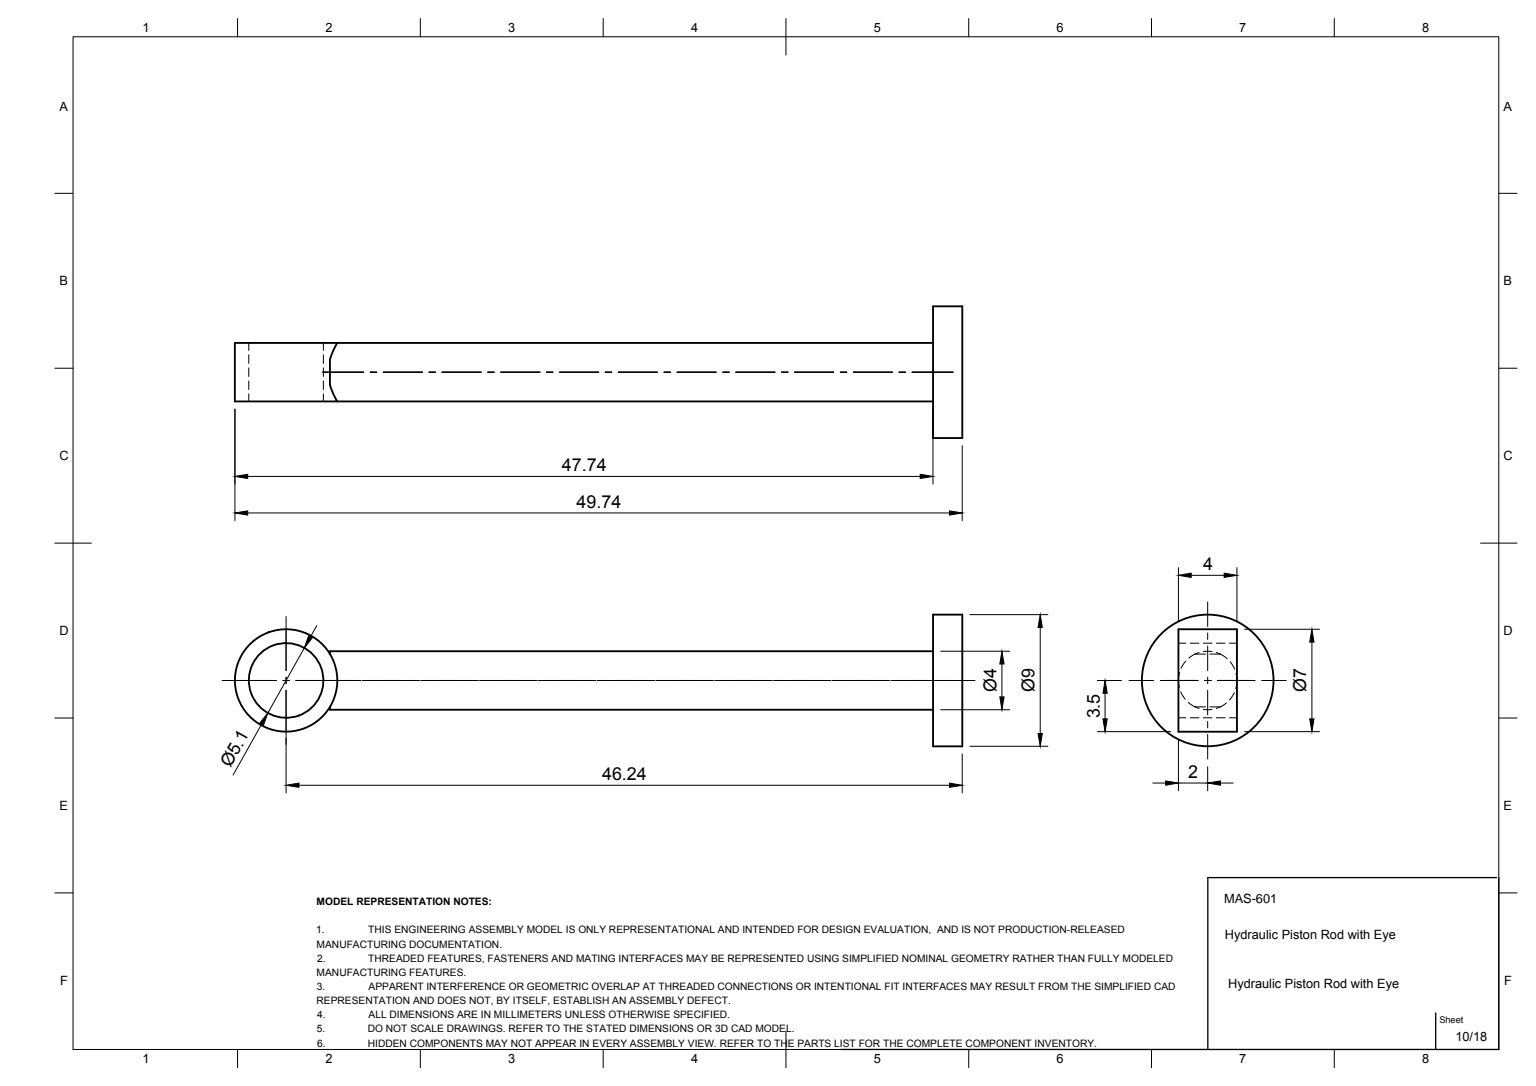
ISO-10303-21;
HEADER;
FILE_DESCRIPTION((''),'2;1');
FILE_NAME('Hydraulic Piston Rod with Eye.step','2026-10-06T07:37:42+05:00',(''),(''),'','','');
FILE_SCHEMA (('AUTOMOTIVE_DESIGN { 1 0 10303 214 3 1 1 }'));
ENDSEC;
DATA;
#10=MECHANICAL_DESIGN_GEOMETRIC_PRESENTATION_REPRESENTATION('',(#378),#18757);
#344=SHAPE_REPRESENTATION_RELATIONSHIP('SRR','None',#18862,#361) ;
#361=ADVANCED_BREP_SHAPE_REPRESENTATION('',(#395),#18745) ;
#378=STYLED_ITEM('',(#18956),#395) ;
#395=MANIFOLD_SOLID_BREP('Hydraulic Piston Rod with Eye',#9547) ;
#424=B_SPLINE_CURVE_WITH_KNOTS('',3,(#14684,#14685,#14686,#14687,#14688,
#14689,#14690,#14691),.UNSPECIFIED.,.F.,.F.,(4,2,2,4),(0.0875095450662273,
0.155297296869045,0.232550630259834,0.309803963650623),.UNSPECIFIED.) ;
#425=B_SPLINE_CURVE_WITH_KNOTS('',3,(#14695,#14696,#14697,#14698,#14699,
#14700,#14701,#14702),.UNSPECIFIED.,.F.,.F.,(4,2,2,4),(0.92941189095187,
1.00666522434266,1.08391855773345,1.15170630953627),.UNSPECIFIED.) ;
#426=B_SPLINE_CURVE_WITH_KNOTS('',3,(#14713,#14714,#14715,#14716,#14717,
#14718,#14719,#14720),.UNSPECIFIED.,.F.,.F.,(4,2,2,4),(0.707117472367471,
0.774905224170291,0.85215855756108,0.92941189095187),.UNSPECIFIED.) ;
#427=B_SPLINE_CURVE_WITH_KNOTS('',3,(#14723,#14724,#14725,#14726,#14727,
#14728,#14729,#14730),.UNSPECIFIED.,.F.,.F.,(4,2,2,4),(0.309803963650623,
0.387057297041413,0.464310630432203,0.532098382235022),.UNSPECIFIED.) ;
#569=CYLINDRICAL_SURFACE('',#10099,3.5) ;
#570=CYLINDRICAL_SURFACE('',#10102,2.55) ;
#571=CYLINDRICAL_SURFACE('',#10105,3.5) ;
#572=CYLINDRICAL_SURFACE('',#10115,2.) ;
#573=CYLINDRICAL_SURFACE('',#10119,4.50000000000001) ;
#717=FACE_BOUND('',#1868,.T.) ;
#718=FACE_BOUND('',#1870,.T.) ;
#719=FACE_BOUND('',#1875,.T.) ;
#862=PLANE('',#10108) ;
#863=PLANE('',#10109) ;
#864=PLANE('',#10110) ;
#865=PLANE('',#10113) ;
#866=PLANE('',#10117) ;
#867=PLANE('',#10121) ;
#1279=FACE_OUTER_BOUND('',#1864,.T.) ;
#1280=FACE_OUTER_BOUND('',#1865,.T.) ;
#1281=FACE_OUTER_BOUND('',#1866,.T.) ;
#1282=FACE_OUTER_BOUND('',#1867,.T.) ;
#1283=FACE_OUTER_BOUND('',#1869,.T.) ;
#1284=FACE_OUTER_BOUND('',#1871,.T.) ;
#1285=FACE_OUTER_BOUND('',#1872,.T.) ;
#1286=FACE_OUTER_BOUND('',#1873,.T.) ;
#1287=FACE_OUTER_BOUND('',#1874,.T.) ;
#1288=FACE_OUTER_BOUND('',#1876,.T.) ;
#1289=FACE_OUTER_BOUND('',#1877,.T.) ;
#1864=EDGE_LOOP('',(#7307,#7308,#7309,#7310,#7311,#7312)) ;
#1865=EDGE_LOOP('',(#7313,#7314,#7315,#7316)) ;
#1866=EDGE_LOOP('',(#7317,#7318,#7319,#7320,#7321,#7322)) ;
#1867=EDGE_LOOP('',(#7323,#7324)) ;
#1868=EDGE_LOOP('',(#7325)) ;
#1869=EDGE_LOOP('',(#7326,#7327)) ;
#1870=EDGE_LOOP('',(#7328)) ;
#1871=EDGE_LOOP('',(#7329,#7330,#7331)) ;
#1872=EDGE_LOOP('',(#7332,#7333)) ;
#1873=EDGE_LOOP('',(#7334,#7335,#7336,#7337,#7338,#7339,#7340,#7341,#7342,
#7343)) ;
#1874=EDGE_LOOP('',(#7344)) ;
#1875=EDGE_LOOP('',(#7345)) ;
#1876=EDGE_LOOP('',(#7346,#7347,#7348,#7349)) ;
#1877=EDGE_LOOP('',(#7350)) ;
#2545=LINE('',#14680,#3316) ;
#2546=LINE('',#14693,#3317) ;
#2547=LINE('',#14708,#3318) ;
#2548=LINE('',#14722,#3319) ;
#2549=LINE('',#14743,#3320) ;
#2550=LINE('',#14750,#3321) ;
#3316=VECTOR('',#11733,3.5) ;
#3317=VECTOR('',#11736,10.) ;
#3318=VECTOR('',#11743,2.55) ;
#3319=VECTOR('',#11750,10.) ;
#3320=VECTOR('',#11771,2.) ;
#3321=VECTOR('',#11780,4.50000000000001) ;
#3928=CIRCLE('',#10100,3.5) ;
#3929=CIRCLE('',#10101,3.5) ;
#3930=CIRCLE('',#10103,2.55) ;
#3931=CIRCLE('',#10104,2.55) ;
#3932=CIRCLE('',#10106,3.5) ;
#3933=CIRCLE('',#10107,3.5) ;
#3934=CIRCLE('',#10111,2.) ;
#3935=CIRCLE('',#10112,2.) ;
#3936=CIRCLE('',#10114,2.) ;
#3937=CIRCLE('',#10116,2.) ;
#3938=CIRCLE('',#10118,4.50000000000001) ;
#3939=CIRCLE('',#10120,4.50000000000001) ;
#4466=VERTEX_POINT('',#14678) ;
#4467=VERTEX_POINT('',#14679) ;
#4468=VERTEX_POINT('',#14681) ;
#4469=VERTEX_POINT('',#14683) ;
#4470=VERTEX_POINT('',#14692) ;
#4471=VERTEX_POINT('',#14694) ;
#4472=VERTEX_POINT('',#14705) ;
#4473=VERTEX_POINT('',#14707) ;
#4474=VERTEX_POINT('',#14712) ;
#4475=VERTEX_POINT('',#14721) ;
#4476=VERTEX_POINT('',#14735) ;
#4477=VERTEX_POINT('',#14741) ;
#4478=VERTEX_POINT('',#14745) ;
#4479=VERTEX_POINT('',#14748) ;
#5500=EDGE_CURVE('',#4466,#4467,#2545,.T.) ;
#5501=EDGE_CURVE('',#4468,#4466,#3928,.T.) ;
#5502=EDGE_CURVE('',#4469,#4468,#424,.T.) ;
#5503=EDGE_CURVE('',#4470,#4469,#2546,.T.) ;
#5504=EDGE_CURVE('',#4471,#4470,#425,.T.) ;
#5505=EDGE_CURVE('',#4471,#4467,#3929,.T.) ;
#5506=EDGE_CURVE('',#4472,#4472,#3930,.T.) ;
#5507=EDGE_CURVE('',#4472,#4473,#2547,.T.) ;
#5508=EDGE_CURVE('',#4473,#4473,#3931,.T.) ;
#5509=EDGE_CURVE('',#4467,#4471,#3932,.T.) ;
#5510=EDGE_CURVE('',#4474,#4471,#426,.T.) ;
#5511=EDGE_CURVE('',#4475,#4474,#2548,.T.) ;
#5512=EDGE_CURVE('',#4468,#4475,#427,.T.) ;
#5513=EDGE_CURVE('',#4466,#4468,#3933,.T.) ;
#5514=EDGE_CURVE('',#4476,#4474,#3934,.T.) ;
#5515=EDGE_CURVE('',#4475,#4476,#3935,.T.) ;
#5516=EDGE_CURVE('',#4470,#4469,#3936,.T.) ;
#5517=EDGE_CURVE('',#4477,#4477,#3937,.T.) ;
#5518=EDGE_CURVE('',#4477,#4476,#2549,.T.) ;
#5519=EDGE_CURVE('',#4478,#4478,#3938,.T.) ;
#5520=EDGE_CURVE('',#4479,#4479,#3939,.T.) ;
#5521=EDGE_CURVE('',#4479,#4478,#2550,.T.) ;
#7307=ORIENTED_EDGE('',*,*,#5500,.F.) ;
#7308=ORIENTED_EDGE('',*,*,#5501,.F.) ;
#7309=ORIENTED_EDGE('',*,*,#5502,.F.) ;
#7310=ORIENTED_EDGE('',*,*,#5503,.F.) ;
#7311=ORIENTED_EDGE('',*,*,#5504,.F.) ;
#7312=ORIENTED_EDGE('',*,*,#5505,.T.) ;
#7313=ORIENTED_EDGE('',*,*,#5506,.F.) ;
#7314=ORIENTED_EDGE('',*,*,#5507,.T.) ;
#7315=ORIENTED_EDGE('',*,*,#5508,.F.) ;
#7316=ORIENTED_EDGE('',*,*,#5507,.F.) ;
#7317=ORIENTED_EDGE('',*,*,#5500,.T.) ;
#7318=ORIENTED_EDGE('',*,*,#5509,.T.) ;
#7319=ORIENTED_EDGE('',*,*,#5510,.F.) ;
#7320=ORIENTED_EDGE('',*,*,#5511,.F.) ;
#7321=ORIENTED_EDGE('',*,*,#5512,.F.) ;
#7322=ORIENTED_EDGE('',*,*,#5513,.F.) ;
#7323=ORIENTED_EDGE('',*,*,#5501,.T.) ;
#7324=ORIENTED_EDGE('',*,*,#5513,.T.) ;
#7325=ORIENTED_EDGE('',*,*,#5508,.T.) ;
#7326=ORIENTED_EDGE('',*,*,#5505,.F.) ;
#7327=ORIENTED_EDGE('',*,*,#5509,.F.) ;
#7328=ORIENTED_EDGE('',*,*,#5506,.T.) ;
#7329=ORIENTED_EDGE('',*,*,#5511,.T.) ;
#7330=ORIENTED_EDGE('',*,*,#5514,.F.) ;
#7331=ORIENTED_EDGE('',*,*,#5515,.F.) ;
#7332=ORIENTED_EDGE('',*,*,#5503,.T.) ;
#7333=ORIENTED_EDGE('',*,*,#5516,.F.) ;
#7334=ORIENTED_EDGE('',*,*,#5517,.F.) ;
#7335=ORIENTED_EDGE('',*,*,#5518,.T.) ;
#7336=ORIENTED_EDGE('',*,*,#5514,.T.) ;
#7337=ORIENTED_EDGE('',*,*,#5510,.T.) ;
#7338=ORIENTED_EDGE('',*,*,#5504,.T.) ;
#7339=ORIENTED_EDGE('',*,*,#5516,.T.) ;
#7340=ORIENTED_EDGE('',*,*,#5502,.T.) ;
#7341=ORIENTED_EDGE('',*,*,#5512,.T.) ;
#7342=ORIENTED_EDGE('',*,*,#5515,.T.) ;
#7343=ORIENTED_EDGE('',*,*,#5518,.F.) ;
#7344=ORIENTED_EDGE('',*,*,#5519,.F.) ;
#7345=ORIENTED_EDGE('',*,*,#5517,.T.) ;
#7346=ORIENTED_EDGE('',*,*,#5520,.F.) ;
#7347=ORIENTED_EDGE('',*,*,#5521,.T.) ;
#7348=ORIENTED_EDGE('',*,*,#5519,.T.) ;
#7349=ORIENTED_EDGE('',*,*,#5521,.F.) ;
#7350=ORIENTED_EDGE('',*,*,#5520,.T.) ;
#9215=ADVANCED_FACE('',(#1279),#569,.T.) ;
#9216=ADVANCED_FACE('',(#1280),#570,.F.) ;
#9217=ADVANCED_FACE('',(#1281),#571,.T.) ;
#9218=ADVANCED_FACE('',(#1282,#717),#862,.T.) ;
#9219=ADVANCED_FACE('',(#1283,#718),#863,.F.) ;
#9220=ADVANCED_FACE('',(#1284),#864,.T.) ;
#9221=ADVANCED_FACE('',(#1285),#865,.T.) ;
#9222=ADVANCED_FACE('',(#1286),#572,.T.) ;
#9223=ADVANCED_FACE('',(#1287,#719),#866,.T.) ;
#9224=ADVANCED_FACE('',(#1288),#573,.T.) ;
#9225=ADVANCED_FACE('',(#1289),#867,.T.) ;
#9547=CLOSED_SHELL('',(#9215,#9216,#9217,#9218,#9219,#9220,#9221,#9222,
#9223,#9224,#9225)) ;
#10098=AXIS2_PLACEMENT_3D('',#14676,#11729,#11730) ;
#10099=AXIS2_PLACEMENT_3D('',#14677,#11731,#11732) ;
#10100=AXIS2_PLACEMENT_3D('',#14682,#11734,#11735) ;
#10101=AXIS2_PLACEMENT_3D('',#14703,#11737,#11738) ;
#10102=AXIS2_PLACEMENT_3D('',#14704,#11739,#11740) ;
#10103=AXIS2_PLACEMENT_3D('',#14706,#11741,#11742) ;
#10104=AXIS2_PLACEMENT_3D('',#14709,#11744,#11745) ;
#10105=AXIS2_PLACEMENT_3D('',#14710,#11746,#11747) ;
#10106=AXIS2_PLACEMENT_3D('',#14711,#11748,#11749) ;
#10107=AXIS2_PLACEMENT_3D('',#14731,#11751,#11752) ;
#10108=AXIS2_PLACEMENT_3D('',#14732,#11753,#11754) ;
#10109=AXIS2_PLACEMENT_3D('',#14733,#11755,#11756) ;
#10110=AXIS2_PLACEMENT_3D('',#14734,#11757,#11758) ;
#10111=AXIS2_PLACEMENT_3D('',#14736,#11759,#11760) ;
#10112=AXIS2_PLACEMENT_3D('',#14737,#11761,#11762) ;
#10113=AXIS2_PLACEMENT_3D('',#14738,#11763,#11764) ;
#10114=AXIS2_PLACEMENT_3D('',#14739,#11765,#11766) ;
#10115=AXIS2_PLACEMENT_3D('',#14740,#11767,#11768) ;
#10116=AXIS2_PLACEMENT_3D('',#14742,#11769,#11770) ;
#10117=AXIS2_PLACEMENT_3D('',#14744,#11772,#11773) ;
#10118=AXIS2_PLACEMENT_3D('',#14746,#11774,#11775) ;
#10119=AXIS2_PLACEMENT_3D('',#14747,#11776,#11777) ;
#10120=AXIS2_PLACEMENT_3D('',#14749,#11778,#11779) ;
#10121=AXIS2_PLACEMENT_3D('',#14751,#11781,#11782) ;
#11729=DIRECTION('axis',(0.,0.,1.)) ;
#11730=DIRECTION('refdir',(1.,0.,0.)) ;
#11731=DIRECTION('center_axis',(0.,1.,0.)) ;
#11732=DIRECTION('ref_axis',(1.,0.,0.)) ;
#11733=DIRECTION('',(0.,-1.,0.)) ;
#11734=DIRECTION('center_axis',(0.,1.,0.)) ;
#11735=DIRECTION('ref_axis',(1.,0.,0.)) ;
#11736=DIRECTION('',(0.,1.,0.)) ;
#11737=DIRECTION('center_axis',(0.,1.,0.)) ;
#11738=DIRECTION('ref_axis',(1.,0.,0.)) ;
#11739=DIRECTION('center_axis',(0.,1.,0.)) ;
#11740=DIRECTION('ref_axis',(1.,0.,0.)) ;
#11741=DIRECTION('center_axis',(0.,1.,0.)) ;
#11742=DIRECTION('ref_axis',(1.,0.,0.)) ;
#11743=DIRECTION('',(0.,1.,0.)) ;
#11744=DIRECTION('center_axis',(0.,-1.,0.)) ;
#11745=DIRECTION('ref_axis',(1.,0.,0.)) ;
#11746=DIRECTION('center_axis',(0.,1.,0.)) ;
#11747=DIRECTION('ref_axis',(1.,0.,0.)) ;
#11748=DIRECTION('center_axis',(0.,1.,0.)) ;
#11749=DIRECTION('ref_axis',(1.,0.,0.)) ;
#11750=DIRECTION('',(0.,-1.,0.)) ;
#11751=DIRECTION('center_axis',(0.,1.,0.)) ;
#11752=DIRECTION('ref_axis',(1.,0.,0.)) ;
#11753=DIRECTION('center_axis',(0.,1.,0.)) ;
#11754=DIRECTION('ref_axis',(1.,0.,0.)) ;
#11755=DIRECTION('center_axis',(0.,1.,0.)) ;
#11756=DIRECTION('ref_axis',(1.,0.,0.)) ;
#11757=DIRECTION('center_axis',(-0.993765553407216,0.,0.11149002135281)) ;
#11758=DIRECTION('ref_axis',(0.11149002135281,0.,0.993765553407216)) ;
#11759=DIRECTION('center_axis',(0.993765553407216,0.,-0.11149002135281)) ;
#11760=DIRECTION('ref_axis',(0.11149002135281,0.,0.993765553407216)) ;
#11761=DIRECTION('center_axis',(0.993765553407216,0.,-0.11149002135281)) ;
#11762=DIRECTION('ref_axis',(0.11149002135281,0.,0.993765553407216)) ;
#11763=DIRECTION('center_axis',(-0.993765553407216,0.,0.11149002135281)) ;
#11764=DIRECTION('ref_axis',(0.11149002135281,0.,0.993765553407216)) ;
#11765=DIRECTION('center_axis',(0.993765553407216,0.,-0.11149002135281)) ;
#11766=DIRECTION('ref_axis',(0.11149002135281,0.,0.993765553407216)) ;
#11767=DIRECTION('center_axis',(0.993765553407216,0.,-0.11149002135281)) ;
#11768=DIRECTION('ref_axis',(-0.111490021352811,0.,-0.993765553407216)) ;
#11769=DIRECTION('center_axis',(0.993765553407216,0.,-0.11149002135281)) ;
#11770=DIRECTION('ref_axis',(0.11149002135281,0.,0.993765553407216)) ;
#11771=DIRECTION('',(-0.993765553407216,0.,0.11149002135281)) ;
#11772=DIRECTION('center_axis',(-0.993765553407216,0.,0.11149002135281)) ;
#11773=DIRECTION('ref_axis',(0.11149002135281,0.,0.993765553407216)) ;
#11774=DIRECTION('center_axis',(0.993765553407216,0.,-0.11149002135281)) ;
#11775=DIRECTION('ref_axis',(0.11149002135281,0.,0.993765553407216)) ;
#11776=DIRECTION('center_axis',(0.993765553407216,0.,-0.11149002135281)) ;
#11777=DIRECTION('ref_axis',(-0.111490021352811,0.,-0.993765553407216)) ;
#11778=DIRECTION('center_axis',(0.993765553407216,0.,-0.11149002135281)) ;
#11779=DIRECTION('ref_axis',(0.11149002135281,0.,0.993765553407216)) ;
#11780=DIRECTION('',(-0.993765553407216,0.,0.11149002135281)) ;
#11781=DIRECTION('center_axis',(0.993765553407216,0.,-0.11149002135281)) ;
#11782=DIRECTION('ref_axis',(-0.11149002135281,0.,-0.993765553407216)) ;
#14676=CARTESIAN_POINT('',(0.,0.,0.)) ;
#14677=CARTESIAN_POINT('Origin',(22.1051760182835,-2.,41.1586206896552)) ;
#14678=CARTESIAN_POINT('',(18.6051760182835,2.00000000000001,41.1586206896552)) ;
#14679=CARTESIAN_POINT('',(18.6051760182835,-2.00000000000001,41.1586206896552)) ;
#14680=CARTESIAN_POINT('',(18.6051760182835,-2.,41.1586206896552)) ;
#14681=CARTESIAN_POINT('',(25.5833554552088,2.,40.7684056149203)) ;
#14682=CARTESIAN_POINT('Origin',(22.1051760182835,2.,41.1586206896552)) ;
#14683=CARTESIAN_POINT('',(24.8854811841601,0.866025403784449,39.032614296297)) ;
#14684=CARTESIAN_POINT('Ctrl Pts',(24.8854811841601,0.866025403784446,39.032614296297)) ;
#14685=CARTESIAN_POINT('Ctrl Pts',(24.9563991705139,1.07434212579119,39.1253579702713)) ;
#14686=CARTESIAN_POINT('Ctrl Pts',(25.0451560272598,1.26170274467392,39.2522326008807)) ;
#14687=CARTESIAN_POINT('Ctrl Pts',(25.2247815177785,1.58802031554125,39.5604452573204)) ;
#14688=CARTESIAN_POINT('Ctrl Pts',(25.3282720606242,1.74115309287314,39.7711453733977)) ;
#14689=CARTESIAN_POINT('Ctrl Pts',(25.4937233402356,1.94729108188327,40.2469283253369)) ;
#14690=CARTESIAN_POINT('Ctrl Pts',(25.5546455359111,2.,40.5124999428882)) ;
#14691=CARTESIAN_POINT('Ctrl Pts',(25.5833554552088,2.00000000000001,40.7684056149203)) ;
#14692=CARTESIAN_POINT('',(24.8854811841601,-0.866025403784449,39.032614296297)) ;
#14693=CARTESIAN_POINT('',(24.8854811841601,-2.,39.032614296297)) ;
#14694=CARTESIAN_POINT('',(25.5833554552088,-2.,40.7684056149203)) ;
#14695=CARTESIAN_POINT('Ctrl Pts',(25.5833554552088,-2.00000000000001,40.7684056149203)) ;
#14696=CARTESIAN_POINT('Ctrl Pts',(25.5546455359111,-2.,40.5124999428882)) ;
#14697=CARTESIAN_POINT('Ctrl Pts',(25.4937233402356,-1.94729108188327,40.2469283253369)) ;
#14698=CARTESIAN_POINT('Ctrl Pts',(25.3282720606242,-1.74115309287314,39.7711453733977)) ;
#14699=CARTESIAN_POINT('Ctrl Pts',(25.2247815177785,-1.58802031554125,39.5604452573204)) ;
#14700=CARTESIAN_POINT('Ctrl Pts',(25.0451560272598,-1.26170274467392,39.2522326008807)) ;
#14701=CARTESIAN_POINT('Ctrl Pts',(24.9563991705139,-1.07434212579119,39.1253579702713)) ;
#14702=CARTESIAN_POINT('Ctrl Pts',(24.8854811841601,-0.866025403784446,
39.032614296297)) ;
#14703=CARTESIAN_POINT('Origin',(22.1051760182835,-2.,41.1586206896552)) ;
#14704=CARTESIAN_POINT('Origin',(22.1051760182835,-2.5,41.1586206896552)) ;
#14705=CARTESIAN_POINT('',(19.5551760182835,-2.,41.1586206896552)) ;
#14706=CARTESIAN_POINT('Origin',(22.1051760182835,-2.,41.1586206896552)) ;
#14707=CARTESIAN_POINT('',(19.5551760182835,2.,41.1586206896552)) ;
#14708=CARTESIAN_POINT('',(19.5551760182835,-2.5,41.1586206896552)) ;
#14709=CARTESIAN_POINT('Origin',(22.1051760182835,2.,41.1586206896552)) ;
#14710=CARTESIAN_POINT('Origin',(22.1051760182835,-2.,41.1586206896552)) ;
#14711=CARTESIAN_POINT('Origin',(22.1051760182835,-2.,41.1586206896552)) ;
#14712=CARTESIAN_POINT('',(25.2874641728502,-0.866025403784418,42.6156869548965)) ;
#14713=CARTESIAN_POINT('Ctrl Pts',(25.2874641728502,-0.866025403784424,
42.6156869548965)) ;
#14714=CARTESIAN_POINT('Ctrl Pts',(25.3360680744367,-1.07434212579117,42.5095341847899)) ;
#14715=CARTESIAN_POINT('Ctrl Pts',(25.3945042964362,-1.26170274467391,42.3661460420789)) ;
#14716=CARTESIAN_POINT('Ctrl Pts',(25.5013674810673,-1.58802031554125,42.0257923757197)) ;
#14717=CARTESIAN_POINT('Ctrl Pts',(25.5555962292677,-1.74115309287314,41.7973978174612)) ;
#14718=CARTESIAN_POINT('Ctrl Pts',(25.6115056919801,-1.94729108188327,41.296780523253)) ;
#14719=CARTESIAN_POINT('Ctrl Pts',(25.6120653745065,-2.,41.0243112869525)) ;
#14720=CARTESIAN_POINT('Ctrl Pts',(25.5833554552088,-1.99999999999999,40.7684056149203)) ;
#14721=CARTESIAN_POINT('',(25.2874641728502,0.866025403784418,42.6156869548965)) ;
#14722=CARTESIAN_POINT('',(25.2874641728502,-2.,42.6156869548965)) ;
#14723=CARTESIAN_POINT('Ctrl Pts',(25.5833554552088,1.99999999999999,40.7684056149203)) ;
#14724=CARTESIAN_POINT('Ctrl Pts',(25.6120653745065,2.,41.0243112869525)) ;
#14725=CARTESIAN_POINT('Ctrl Pts',(25.6115056919801,1.94729108188327,41.296780523253)) ;
#14726=CARTESIAN_POINT('Ctrl Pts',(25.5555962292677,1.74115309287314,41.7973978174612)) ;
#14727=CARTESIAN_POINT('Ctrl Pts',(25.5013674810673,1.58802031554125,42.0257923757197)) ;
#14728=CARTESIAN_POINT('Ctrl Pts',(25.3945042964362,1.26170274467391,42.3661460420789)) ;
#14729=CARTESIAN_POINT('Ctrl Pts',(25.3360680744367,1.07434212579117,42.5095341847899)) ;
#14730=CARTESIAN_POINT('Ctrl Pts',(25.2874641728502,0.866025403784424,42.6156869548965)) ;
#14731=CARTESIAN_POINT('Origin',(22.1051760182835,2.,41.1586206896552)) ;
#14732=CARTESIAN_POINT('Origin',(22.1051760182835,2.,41.1586206896552)) ;
#14733=CARTESIAN_POINT('Origin',(22.1051760182835,-2.,41.1586206896552)) ;
#14734=CARTESIAN_POINT('Origin',(24.8634926357996,0.,38.8366195187823)) ;
#14735=CARTESIAN_POINT('',(25.3094527212108,-2.44929359829471E-16,42.8116817324112)) ;
#14736=CARTESIAN_POINT('Origin',(25.0864726785052,0.,40.8241506255967)) ;
#14737=CARTESIAN_POINT('Origin',(25.0864726785052,0.,40.8241506255967)) ;
#14738=CARTESIAN_POINT('Origin',(24.8634926357996,0.,38.8366195187823)) ;
#14739=CARTESIAN_POINT('Origin',(25.0864726785052,0.,40.8241506255967)) ;
#14740=CARTESIAN_POINT('Origin',(45.5775257955129,0.,38.5252704302388)) ;
#14741=CARTESIAN_POINT('',(66.2915589552262,-2.44929359829471E-16,38.2139213416953)) ;
#14742=CARTESIAN_POINT('Origin',(66.0685789125206,0.,36.2263902348809)) ;
#14743=CARTESIAN_POINT('',(45.8005058382185,-2.44929359829471E-16,40.5128015370533)) ;
#14744=CARTESIAN_POINT('Origin',(65.566873816433,0.,31.7544452445484)) ;
#14745=CARTESIAN_POINT('',(66.5702840086083,-5.5109105961631E-16,40.6983352252134)) ;
#14746=CARTESIAN_POINT('Origin',(66.0685789125206,0.,36.2263902348809)) ;
#14747=CARTESIAN_POINT('Origin',(67.0623444659278,0.,36.1149002135281)) ;
#14748=CARTESIAN_POINT('',(68.5578151154227,-5.5109105961631E-16,40.4753551825078)) ;
#14749=CARTESIAN_POINT('Origin',(68.0561100193351,0.,36.0034101921753)) ;
#14750=CARTESIAN_POINT('',(67.5640495620155,-5.5109105961631E-16,40.5868452038606)) ;
#14751=CARTESIAN_POINT('Origin',(68.0561100193351,0.,36.0034101921753)) ;
#18726=UNCERTAINTY_MEASURE_WITH_UNIT(LENGTH_MEASURE(0.01),#18758,
'DISTANCE_ACCURACY_VALUE',
'Maximum model space distance between geometric entities at asserted c
onnectivities') ;
#18738=UNCERTAINTY_MEASURE_WITH_UNIT(LENGTH_MEASURE(0.01),#18758,
'DISTANCE_ACCURACY_VALUE',
'Maximum model space distance between geometric entities at asserted c
onnectivities') ;
#18745=(
GEOMETRIC_REPRESENTATION_CONTEXT(3)
GLOBAL_UNCERTAINTY_ASSIGNED_CONTEXT((#18726))
GLOBAL_UNIT_ASSIGNED_CONTEXT((#18758,#18760,#18761))
REPRESENTATION_CONTEXT('','3D')
) ;
#18757=(
GEOMETRIC_REPRESENTATION_CONTEXT(3)
GLOBAL_UNCERTAINTY_ASSIGNED_CONTEXT((#18738))
GLOBAL_UNIT_ASSIGNED_CONTEXT((#18758,#18760,#18761))
REPRESENTATION_CONTEXT('','3D')
) ;
#18758=(
LENGTH_UNIT()
NAMED_UNIT(*)
SI_UNIT(.MILLI.,.METRE.)
) ;
#18760=(
NAMED_UNIT(*)
PLANE_ANGLE_UNIT()
SI_UNIT($,.RADIAN.)
) ;
#18761=(
NAMED_UNIT(*)
SI_UNIT($,.STERADIAN.)
SOLID_ANGLE_UNIT()
) ;
#18768=SHAPE_DEFINITION_REPRESENTATION(#18786,#18862) ;
#18786=PRODUCT_DEFINITION_SHAPE('',$,#18881) ;
#18862=SHAPE_REPRESENTATION('',(#10098),#18745) ;
#18874=PRODUCT_DEFINITION_CONTEXT('part definition',#18930,'design') ;
#18881=PRODUCT_DEFINITION('Hydraulic Piston Rod with Eye',
'Hydraulic Piston Rod with Eye',#18899,#18874) ;
#18899=PRODUCT_DEFINITION_FORMATION('',$,#18938) ;
#18930=APPLICATION_CONTEXT(
'Core Data for Automotive Mechanical Design Process') ;
#18931=PRODUCT_CONTEXT('part definition',#18930,'mechanical') ;
#18938=PRODUCT('Hydraulic Piston Rod with Eye',
'Hydraulic Piston Rod with Eye',$,(#18931)) ;
#18956=PRESENTATION_STYLE_ASSIGNMENT((#18974)) ;
#18974=SURFACE_STYLE_USAGE(.BOTH.,#18992) ;
#18992=SURFACE_SIDE_STYLE('',(#19010)) ;
#19010=SURFACE_STYLE_FILL_AREA(#19028) ;
#19028=FILL_AREA_STYLE(
'MAS-253 Metallic Sheet - Hydraulic Piston Rod with Eye',(#19046)) ;
#19046=FILL_AREA_STYLE_COLOUR(
'MAS-253 Metallic Sheet - Hydraulic Piston Rod with Eye',#19064) ;
#19064=COLOUR_RGB(
'MAS-253 Metallic Sheet - Hydraulic Piston Rod with Eye', 0.09019608, 0.27058824, 0.51372549) ;
ENDSEC;
END-ISO-10303-21;
